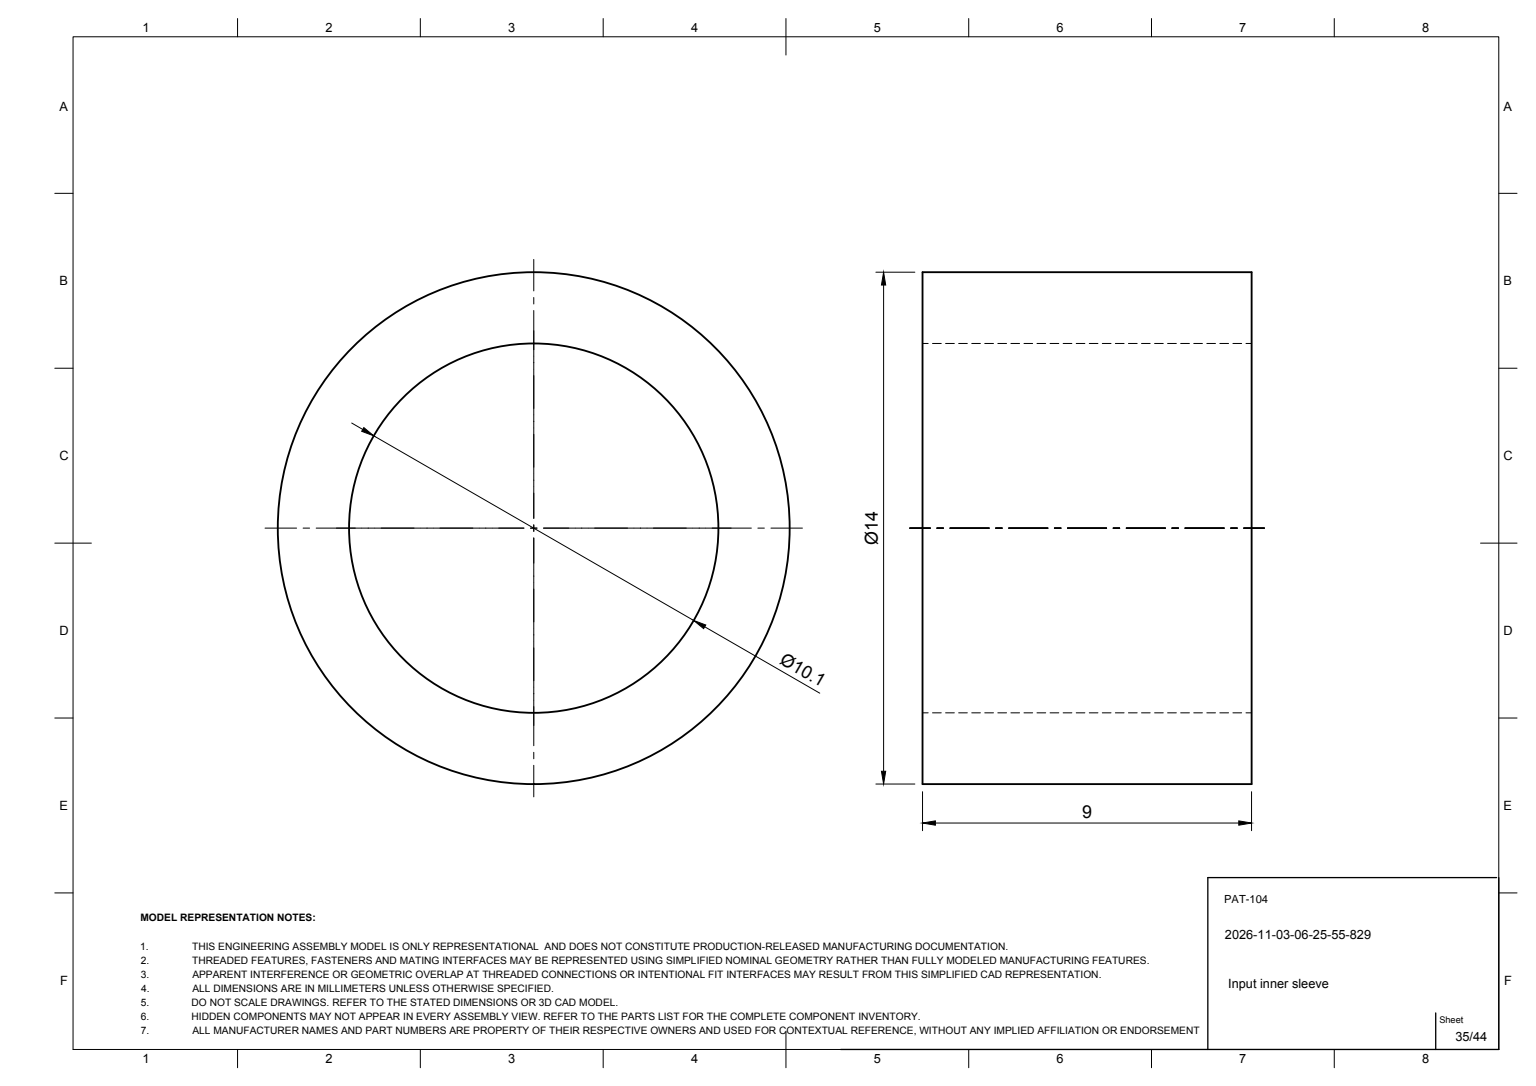
ISO-10303-21;
HEADER;
/* Generated by software containing ST-Developer
 * from STEP Tools, Inc. (www.steptools.com) 
 */

FILE_DESCRIPTION(
/* description */ ('Timing belt drive module 2 mm Pitch Timing 20T-40T'),

/* implementation_level */ '2;1');

FILE_NAME(
/* name */ 'Input inner sleeve.step',
/* time_stamp */ '2026-10-28T03:25:12-07:00',
/* author */ (''),
/* organization */ (''),
/* preprocessor_version */ 'ST-DEVELOPER v20.2',
/* originating_system */ 'Autodesk Translation Framework v15.17.0.0',
/* authorisation */ '');

FILE_SCHEMA (('AUTOMOTIVE_DESIGN { 1 0 10303 214 3 1 1 }'));
ENDSEC;

DATA;
#10=MECHANICAL_DESIGN_GEOMETRIC_PRESENTATION_REPRESENTATION('',(#569),#17830);
#468=SHAPE_REPRESENTATION_RELATIONSHIP('SRR','None',#18041,#511);
#511=ADVANCED_BREP_SHAPE_REPRESENTATION('',(#625),#17816);
#569=STYLED_ITEM('',(#18303),#625);
#625=MANIFOLD_SOLID_BREP('Body1',#9028);
#737=FACE_BOUND('',#1903,.T.);
#738=FACE_BOUND('',#1905,.T.);
#918=PLANE('',#10235);
#919=PLANE('',#10236);
#1279=FACE_OUTER_BOUND('',#1900,.T.);
#1280=FACE_OUTER_BOUND('',#1901,.T.);
#1281=FACE_OUTER_BOUND('',#1902,.T.);
#1282=FACE_OUTER_BOUND('',#1904,.T.);
#1900=EDGE_LOOP('',(#7129,#7130,#7131,#7132));
#1901=EDGE_LOOP('',(#7133,#7134,#7135,#7136));
#1902=EDGE_LOOP('',(#7137));
#1903=EDGE_LOOP('',(#7138));
#1904=EDGE_LOOP('',(#7139));
#1905=EDGE_LOOP('',(#7140));
#2490=CIRCLE('',#10230,0.505);
#2491=CIRCLE('',#10231,0.505);
#2492=CIRCLE('',#10233,0.7);
#2493=CIRCLE('',#10234,0.7);
#3086=LINE('',#16017,#3564);
#3087=LINE('',#16023,#3565);
#3564=VECTOR('',#12535,0.505);
#3565=VECTOR('',#12542,0.7);
#4213=VERTEX_POINT('',#16014);
#4214=VERTEX_POINT('',#16016);
#4215=VERTEX_POINT('',#16020);
#4216=VERTEX_POINT('',#16022);
#5247=EDGE_CURVE('',#4213,#4213,#2490,.T.);
#5248=EDGE_CURVE('',#4213,#4214,#3086,.T.);
#5249=EDGE_CURVE('',#4214,#4214,#2491,.T.);
#5250=EDGE_CURVE('',#4215,#4215,#2492,.T.);
#5251=EDGE_CURVE('',#4215,#4216,#3087,.T.);
#5252=EDGE_CURVE('',#4216,#4216,#2493,.T.);
#7129=ORIENTED_EDGE('',*,*,#5247,.F.);
#7130=ORIENTED_EDGE('',*,*,#5248,.T.);
#7131=ORIENTED_EDGE('',*,*,#5249,.T.);
#7132=ORIENTED_EDGE('',*,*,#5248,.F.);
#7133=ORIENTED_EDGE('',*,*,#5250,.F.);
#7134=ORIENTED_EDGE('',*,*,#5251,.T.);
#7135=ORIENTED_EDGE('',*,*,#5252,.T.);
#7136=ORIENTED_EDGE('',*,*,#5251,.F.);
#7137=ORIENTED_EDGE('',*,*,#5250,.T.);
#7138=ORIENTED_EDGE('',*,*,#5247,.T.);
#7139=ORIENTED_EDGE('',*,*,#5252,.F.);
#7140=ORIENTED_EDGE('',*,*,#5249,.F.);
#8304=CYLINDRICAL_SURFACE('',#10229,0.505);
#8305=CYLINDRICAL_SURFACE('',#10232,0.7);
#8777=ADVANCED_FACE('',(#1279),#8304,.F.);
#8778=ADVANCED_FACE('',(#1280),#8305,.T.);
#8779=ADVANCED_FACE('',(#1281,#737),#918,.T.);
#8780=ADVANCED_FACE('',(#1282,#738),#919,.F.);
#9028=CLOSED_SHELL('',(#8777,#8778,#8779,#8780));
#10228=AXIS2_PLACEMENT_3D('',#16012,#12529,#12530);
#10229=AXIS2_PLACEMENT_3D('',#16013,#12531,#12532);
#10230=AXIS2_PLACEMENT_3D('',#16015,#12533,#12534);
#10231=AXIS2_PLACEMENT_3D('',#16018,#12536,#12537);
#10232=AXIS2_PLACEMENT_3D('',#16019,#12538,#12539);
#10233=AXIS2_PLACEMENT_3D('',#16021,#12540,#12541);
#10234=AXIS2_PLACEMENT_3D('',#16024,#12543,#12544);
#10235=AXIS2_PLACEMENT_3D('',#16025,#12545,#12546);
#10236=AXIS2_PLACEMENT_3D('',#16026,#12547,#12548);
#12529=DIRECTION('axis',(0.,0.,1.));
#12530=DIRECTION('refdir',(1.,0.,0.));
#12531=DIRECTION('center_axis',(0.,1.,0.));
#12532=DIRECTION('ref_axis',(1.,0.,0.));
#12533=DIRECTION('center_axis',(0.,-1.,0.));
#12534=DIRECTION('ref_axis',(1.,0.,0.));
#12535=DIRECTION('',(0.,-1.,0.));
#12536=DIRECTION('center_axis',(0.,-1.,0.));
#12537=DIRECTION('ref_axis',(1.,0.,0.));
#12538=DIRECTION('center_axis',(0.,1.,0.));
#12539=DIRECTION('ref_axis',(1.,0.,0.));
#12540=DIRECTION('center_axis',(0.,1.,0.));
#12541=DIRECTION('ref_axis',(1.,0.,0.));
#12542=DIRECTION('',(0.,-1.,0.));
#12543=DIRECTION('center_axis',(0.,1.,0.));
#12544=DIRECTION('ref_axis',(1.,0.,0.));
#12545=DIRECTION('center_axis',(0.,1.,0.));
#12546=DIRECTION('ref_axis',(1.,0.,0.));
#12547=DIRECTION('center_axis',(0.,1.,0.));
#12548=DIRECTION('ref_axis',(1.,0.,0.));
#16012=CARTESIAN_POINT('',(0.,0.,0.));
#16013=CARTESIAN_POINT('Origin',(0.,-0.45,7.));
#16014=CARTESIAN_POINT('',(-0.505,0.45,7.));
#16015=CARTESIAN_POINT('Origin',(0.,0.45,7.));
#16016=CARTESIAN_POINT('',(-0.505,-0.45,7.));
#16017=CARTESIAN_POINT('',(-0.505,-0.45,7.));
#16018=CARTESIAN_POINT('Origin',(0.,-0.45,7.));
#16019=CARTESIAN_POINT('Origin',(0.,-0.45,7.));
#16020=CARTESIAN_POINT('',(-0.7,0.45,7.));
#16021=CARTESIAN_POINT('Origin',(0.,0.45,7.));
#16022=CARTESIAN_POINT('',(-0.7,-0.45,7.));
#16023=CARTESIAN_POINT('',(-0.7,-0.45,7.));
#16024=CARTESIAN_POINT('Origin',(0.,-0.45,7.));
#16025=CARTESIAN_POINT('Origin',(0.,0.45,7.));
#16026=CARTESIAN_POINT('Origin',(0.,-0.45,7.));
#17766=UNCERTAINTY_MEASURE_WITH_UNIT(LENGTH_MEASURE(0.001),#17831,
'DISTANCE_ACCURACY_VALUE',
'Maximum model space distance between geometric entities at asserted c
onnectivities');
#17780=UNCERTAINTY_MEASURE_WITH_UNIT(LENGTH_MEASURE(0.001),#17831,
'DISTANCE_ACCURACY_VALUE',
'Maximum model space distance between geometric entities at asserted c
onnectivities');
#17816=(
GEOMETRIC_REPRESENTATION_CONTEXT(3)
GLOBAL_UNCERTAINTY_ASSIGNED_CONTEXT((#17766))
GLOBAL_UNIT_ASSIGNED_CONTEXT((#17831,#17833,#17834))
REPRESENTATION_CONTEXT('','3D')
);
#17830=(
GEOMETRIC_REPRESENTATION_CONTEXT(3)
GLOBAL_UNCERTAINTY_ASSIGNED_CONTEXT((#17780))
GLOBAL_UNIT_ASSIGNED_CONTEXT((#17831,#17833,#17834))
REPRESENTATION_CONTEXT('','3D')
);
#17831=(
LENGTH_UNIT()
NAMED_UNIT(*)
SI_UNIT(.CENTI.,.METRE.)
);
#17833=(
NAMED_UNIT(*)
PLANE_ANGLE_UNIT()
SI_UNIT($,.RADIAN.)
);
#17834=(
NAMED_UNIT(*)
SI_UNIT($,.STERADIAN.)
SOLID_ANGLE_UNIT()
);
#17870=SHAPE_DEFINITION_REPRESENTATION(#17929,#18041);
#17929=PRODUCT_DEFINITION_SHAPE('',$,#18091);
#18041=SHAPE_REPRESENTATION('',(#10228),#17816);
#18055=PRODUCT_DEFINITION_CONTEXT('part definition',#18204,'design');
#18091=PRODUCT_DEFINITION('Input inner sleeve','Input inner sleeve',#18140,
#18055);
#18140=PRODUCT_DEFINITION_FORMATION('',$,#18241);
#18204=APPLICATION_CONTEXT(
'Core Data for Automotive Mechanical Design Process');
#18205=PRODUCT_CONTEXT('part definition',#18204,'mechanical');
#18241=PRODUCT('Input inner sleeve','Input inner sleeve',
'Input inner sleeve',(#18205));
#18297=COLOUR_RGB('Light Blue',0.38,0.62,0.78);
#18298=FILL_AREA_STYLE_COLOUR('',#18297);
#18299=FILL_AREA_STYLE('',(#18298));
#18300=SURFACE_STYLE_FILL_AREA(#18299);
#18301=SURFACE_SIDE_STYLE('',(#18300));
#18302=SURFACE_STYLE_USAGE(.BOTH.,#18301);
#18303=PRESENTATION_STYLE_ASSIGNMENT((#18302));
ENDSEC;
END-ISO-10303-21;
